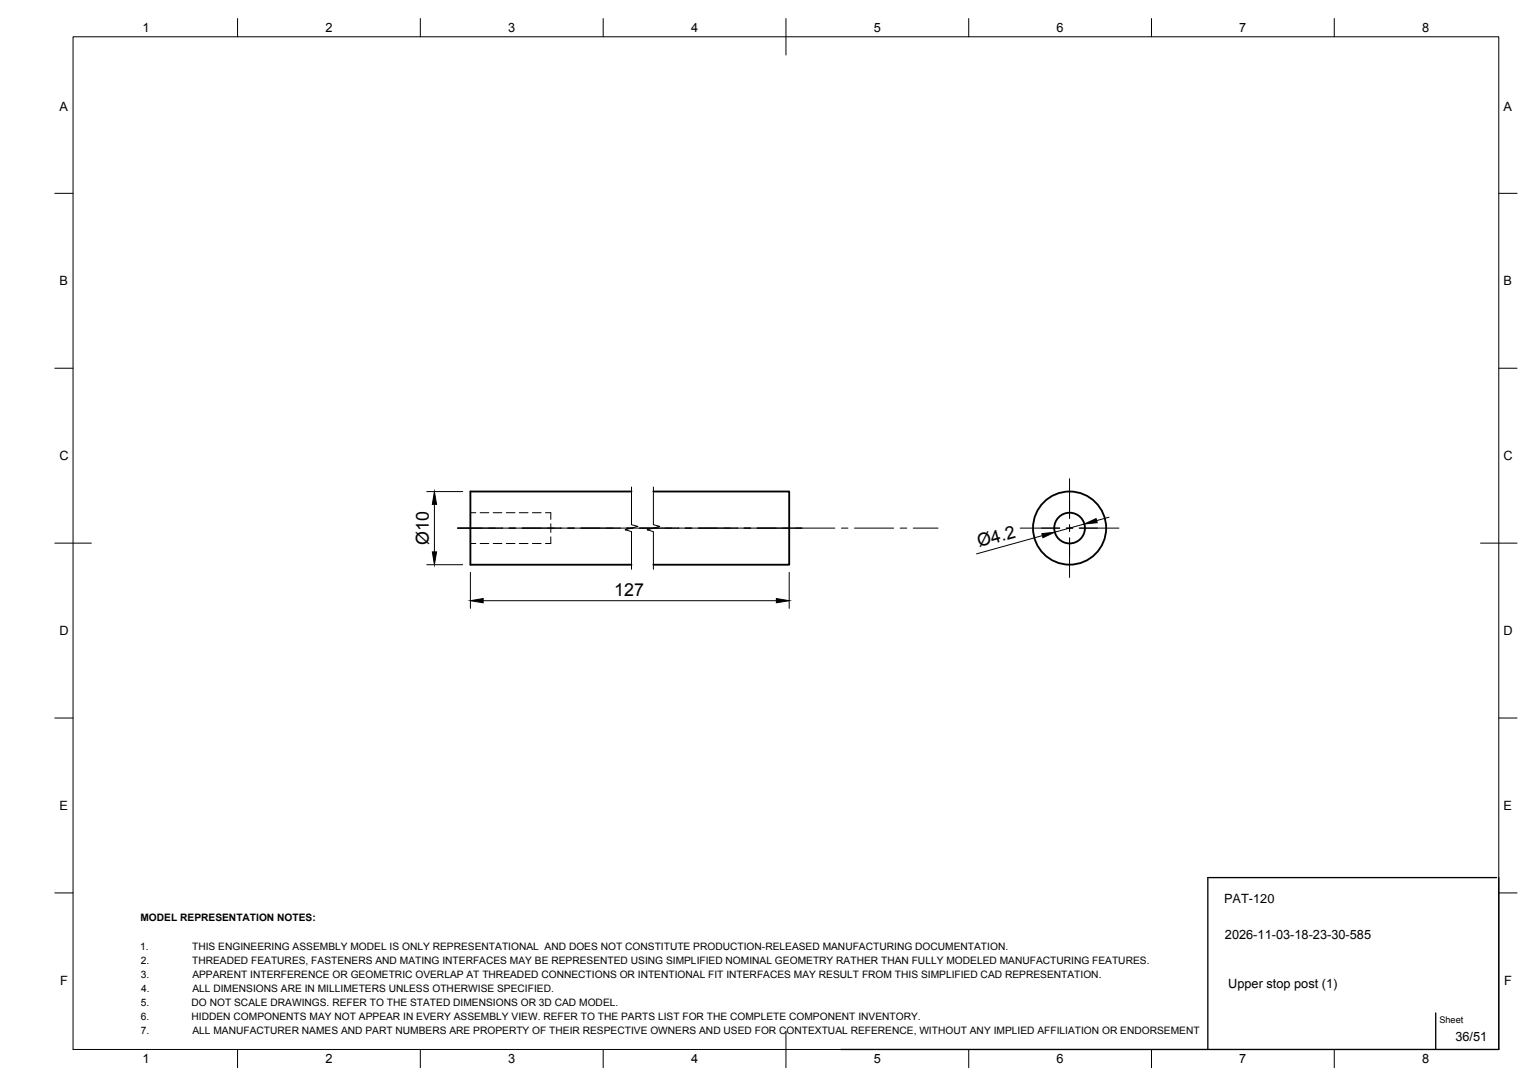
ISO-10303-21;
HEADER;
/* Generated by software containing ST-Developer
 * from STEP Tools, Inc. (www.steptools.com) 
 */

FILE_DESCRIPTION(
/* description */ ('Vibration shaker table dummy'),
/* implementation_level */ '2;1');

FILE_NAME(
/* name */ 'Upper stop post (1).step',
/* time_stamp */ '2026-10-27T10:55:14-07:00',
/* author */ (''),
/* organization */ (''),
/* preprocessor_version */ 'ST-DEVELOPER v20.2',
/* originating_system */ 'Autodesk Translation Framework v15.17.0.0',
/* authorisation */ '');

FILE_SCHEMA (('AUTOMOTIVE_DESIGN { 1 0 10303 214 3 1 1 }'));
ENDSEC;

DATA;
#10=MECHANICAL_DESIGN_GEOMETRIC_PRESENTATION_REPRESENTATION('',(#717),#22394);
#625=SHAPE_REPRESENTATION_RELATIONSHIP('SRR','None',#22671,#671);
#671=ADVANCED_BREP_SHAPE_REPRESENTATION('',(#763),#22377);
#717=STYLED_ITEM('',(#22975),#763);
#763=MANIFOLD_SOLID_BREP('Body1',#9235);
#946=FACE_BOUND('',#2298,.T.);
#1227=PLANE('',#10327);
#1228=PLANE('',#10331);
#1229=PLANE('',#10332);
#1625=FACE_OUTER_BOUND('',#2294,.T.);
#1626=FACE_OUTER_BOUND('',#2295,.T.);
#1627=FACE_OUTER_BOUND('',#2296,.T.);
#1628=FACE_OUTER_BOUND('',#2297,.T.);
#1629=FACE_OUTER_BOUND('',#2299,.T.);
#2294=EDGE_LOOP('',(#7476,#7477,#7478,#7479));
#2295=EDGE_LOOP('',(#7480));
#2296=EDGE_LOOP('',(#7481,#7482,#7483,#7484));
#2297=EDGE_LOOP('',(#7485));
#2298=EDGE_LOOP('',(#7486));
#2299=EDGE_LOOP('',(#7487));
#2983=LINE('',#21074,#3602);
#2984=LINE('',#21081,#3603);
#3602=VECTOR('',#12443,0.21);
#3603=VECTOR('',#12452,0.5);
#4110=CIRCLE('',#10325,0.21);
#4111=CIRCLE('',#10326,0.21);
#4112=CIRCLE('',#10329,0.5);
#4113=CIRCLE('',#10330,0.5);
#4777=VERTEX_POINT('',#21071);
#4778=VERTEX_POINT('',#21073);
#4779=VERTEX_POINT('',#21078);
#4780=VERTEX_POINT('',#21080);
#5731=EDGE_CURVE('',#4777,#4777,#4110,.T.);
#5732=EDGE_CURVE('',#4777,#4778,#2983,.T.);
#5733=EDGE_CURVE('',#4778,#4778,#4111,.T.);
#5734=EDGE_CURVE('',#4779,#4779,#4112,.T.);
#5735=EDGE_CURVE('',#4779,#4780,#2984,.T.);
#5736=EDGE_CURVE('',#4780,#4780,#4113,.T.);
#7476=ORIENTED_EDGE('',*,*,#5731,.F.);
#7477=ORIENTED_EDGE('',*,*,#5732,.T.);
#7478=ORIENTED_EDGE('',*,*,#5733,.F.);
#7479=ORIENTED_EDGE('',*,*,#5732,.F.);
#7480=ORIENTED_EDGE('',*,*,#5731,.T.);
#7481=ORIENTED_EDGE('',*,*,#5734,.F.);
#7482=ORIENTED_EDGE('',*,*,#5735,.T.);
#7483=ORIENTED_EDGE('',*,*,#5736,.T.);
#7484=ORIENTED_EDGE('',*,*,#5735,.F.);
#7485=ORIENTED_EDGE('',*,*,#5734,.T.);
#7486=ORIENTED_EDGE('',*,*,#5733,.T.);
#7487=ORIENTED_EDGE('',*,*,#5736,.F.);
#8619=CYLINDRICAL_SURFACE('',#10324,0.21);
#8620=CYLINDRICAL_SURFACE('',#10328,0.5);
#8990=ADVANCED_FACE('',(#1625),#8619,.F.);
#8991=ADVANCED_FACE('',(#1626),#1227,.T.);
#8992=ADVANCED_FACE('',(#1627),#8620,.T.);
#8993=ADVANCED_FACE('',(#1628,#946),#1228,.T.);
#8994=ADVANCED_FACE('',(#1629),#1229,.F.);
#9235=CLOSED_SHELL('',(#8990,#8991,#8992,#8993,#8994));
#10323=AXIS2_PLACEMENT_3D('',#21069,#12437,#12438);
#10324=AXIS2_PLACEMENT_3D('',#21070,#12439,#12440);
#10325=AXIS2_PLACEMENT_3D('',#21072,#12441,#12442);
#10326=AXIS2_PLACEMENT_3D('',#21075,#12444,#12445);
#10327=AXIS2_PLACEMENT_3D('',#21076,#12446,#12447);
#10328=AXIS2_PLACEMENT_3D('',#21077,#12448,#12449);
#10329=AXIS2_PLACEMENT_3D('',#21079,#12450,#12451);
#10330=AXIS2_PLACEMENT_3D('',#21082,#12453,#12454);
#10331=AXIS2_PLACEMENT_3D('',#21083,#12455,#12456);
#10332=AXIS2_PLACEMENT_3D('',#21084,#12457,#12458);
#12437=DIRECTION('axis',(0.,0.,1.));
#12438=DIRECTION('refdir',(1.,0.,0.));
#12439=DIRECTION('center_axis',(0.,0.,1.));
#12440=DIRECTION('ref_axis',(1.,0.,0.));
#12441=DIRECTION('center_axis',(0.,0.,1.));
#12442=DIRECTION('ref_axis',(1.,0.,0.));
#12443=DIRECTION('',(0.,0.,1.));
#12444=DIRECTION('center_axis',(0.,0.,-1.));
#12445=DIRECTION('ref_axis',(1.,0.,0.));
#12446=DIRECTION('center_axis',(0.,0.,1.));
#12447=DIRECTION('ref_axis',(1.,0.,0.));
#12448=DIRECTION('center_axis',(0.,0.,1.));
#12449=DIRECTION('ref_axis',(1.,0.,0.));
#12450=DIRECTION('center_axis',(0.,0.,1.));
#12451=DIRECTION('ref_axis',(1.,0.,0.));
#12452=DIRECTION('',(0.,0.,-1.));
#12453=DIRECTION('center_axis',(0.,0.,1.));
#12454=DIRECTION('ref_axis',(1.,0.,0.));
#12455=DIRECTION('center_axis',(0.,0.,1.));
#12456=DIRECTION('ref_axis',(1.,0.,0.));
#12457=DIRECTION('center_axis',(0.,0.,1.));
#12458=DIRECTION('ref_axis',(1.,0.,0.));
#21069=CARTESIAN_POINT('',(0.,0.,0.));
#21070=CARTESIAN_POINT('Origin',(0.,6.,29.4));
#21071=CARTESIAN_POINT('',(-0.21,6.,29.4));
#21072=CARTESIAN_POINT('Origin',(0.,6.,29.4));
#21073=CARTESIAN_POINT('',(-0.21,6.,30.5));
#21074=CARTESIAN_POINT('',(-0.21,6.,29.4));
#21075=CARTESIAN_POINT('Origin',(0.,6.,30.5));
#21076=CARTESIAN_POINT('Origin',(0.,6.,29.4));
#21077=CARTESIAN_POINT('Origin',(0.,6.,17.8));
#21078=CARTESIAN_POINT('',(-0.5,6.,30.5));
#21079=CARTESIAN_POINT('Origin',(0.,6.,30.5));
#21080=CARTESIAN_POINT('',(-0.5,6.,17.8));
#21081=CARTESIAN_POINT('',(-0.5,6.,17.8));
#21082=CARTESIAN_POINT('Origin',(0.,6.,17.8));
#21083=CARTESIAN_POINT('Origin',(0.,6.,30.5));
#21084=CARTESIAN_POINT('Origin',(0.,6.,17.8));
#22326=UNCERTAINTY_MEASURE_WITH_UNIT(LENGTH_MEASURE(0.001),#22395,
'DISTANCE_ACCURACY_VALUE',
'Maximum model space distance between geometric entities at asserted c
onnectivities');
#22343=UNCERTAINTY_MEASURE_WITH_UNIT(LENGTH_MEASURE(0.001),#22395,
'DISTANCE_ACCURACY_VALUE',
'Maximum model space distance between geometric entities at asserted c
onnectivities');
#22377=(
GEOMETRIC_REPRESENTATION_CONTEXT(3)
GLOBAL_UNCERTAINTY_ASSIGNED_CONTEXT((#22326))
GLOBAL_UNIT_ASSIGNED_CONTEXT((#22395,#22397,#22398))
REPRESENTATION_CONTEXT('','3D')
);
#22394=(
GEOMETRIC_REPRESENTATION_CONTEXT(3)
GLOBAL_UNCERTAINTY_ASSIGNED_CONTEXT((#22343))
GLOBAL_UNIT_ASSIGNED_CONTEXT((#22395,#22397,#22398))
REPRESENTATION_CONTEXT('','3D')
);
#22395=(
LENGTH_UNIT()
NAMED_UNIT(*)
SI_UNIT(.CENTI.,.METRE.)
);
#22397=(
NAMED_UNIT(*)
PLANE_ANGLE_UNIT()
SI_UNIT($,.RADIAN.)
);
#22398=(
NAMED_UNIT(*)
SI_UNIT($,.STERADIAN.)
SOLID_ANGLE_UNIT()
);
#22432=SHAPE_DEFINITION_REPRESENTATION(#22482,#22671);
#22482=PRODUCT_DEFINITION_SHAPE('',$,#22722);
#22671=SHAPE_REPRESENTATION('',(#10323),#22377);
#22688=PRODUCT_DEFINITION_CONTEXT('part definition',#22840,'design');
#22722=PRODUCT_DEFINITION('Upper stop post (1)','Upper stop post (1)',#22772,
#22688);
#22772=PRODUCT_DEFINITION_FORMATION('',$,#22875);
#22840=APPLICATION_CONTEXT(
'Core Data for Automotive Mechanical Design Process');
#22841=PRODUCT_CONTEXT('part definition',#22840,'mechanical');
#22875=PRODUCT('Upper stop post (1)','Upper stop post (1)',
'Upper stop post (1)',(#22841));
#22969=COLOUR_RGB('Off White',0.89,0.88,0.83);
#22970=FILL_AREA_STYLE_COLOUR('',#22969);
#22971=FILL_AREA_STYLE('',(#22970));
#22972=SURFACE_STYLE_FILL_AREA(#22971);
#22973=SURFACE_SIDE_STYLE('',(#22972));
#22974=SURFACE_STYLE_USAGE(.BOTH.,#22973);
#22975=PRESENTATION_STYLE_ASSIGNMENT((#22974));
ENDSEC;
END-ISO-10303-21;
